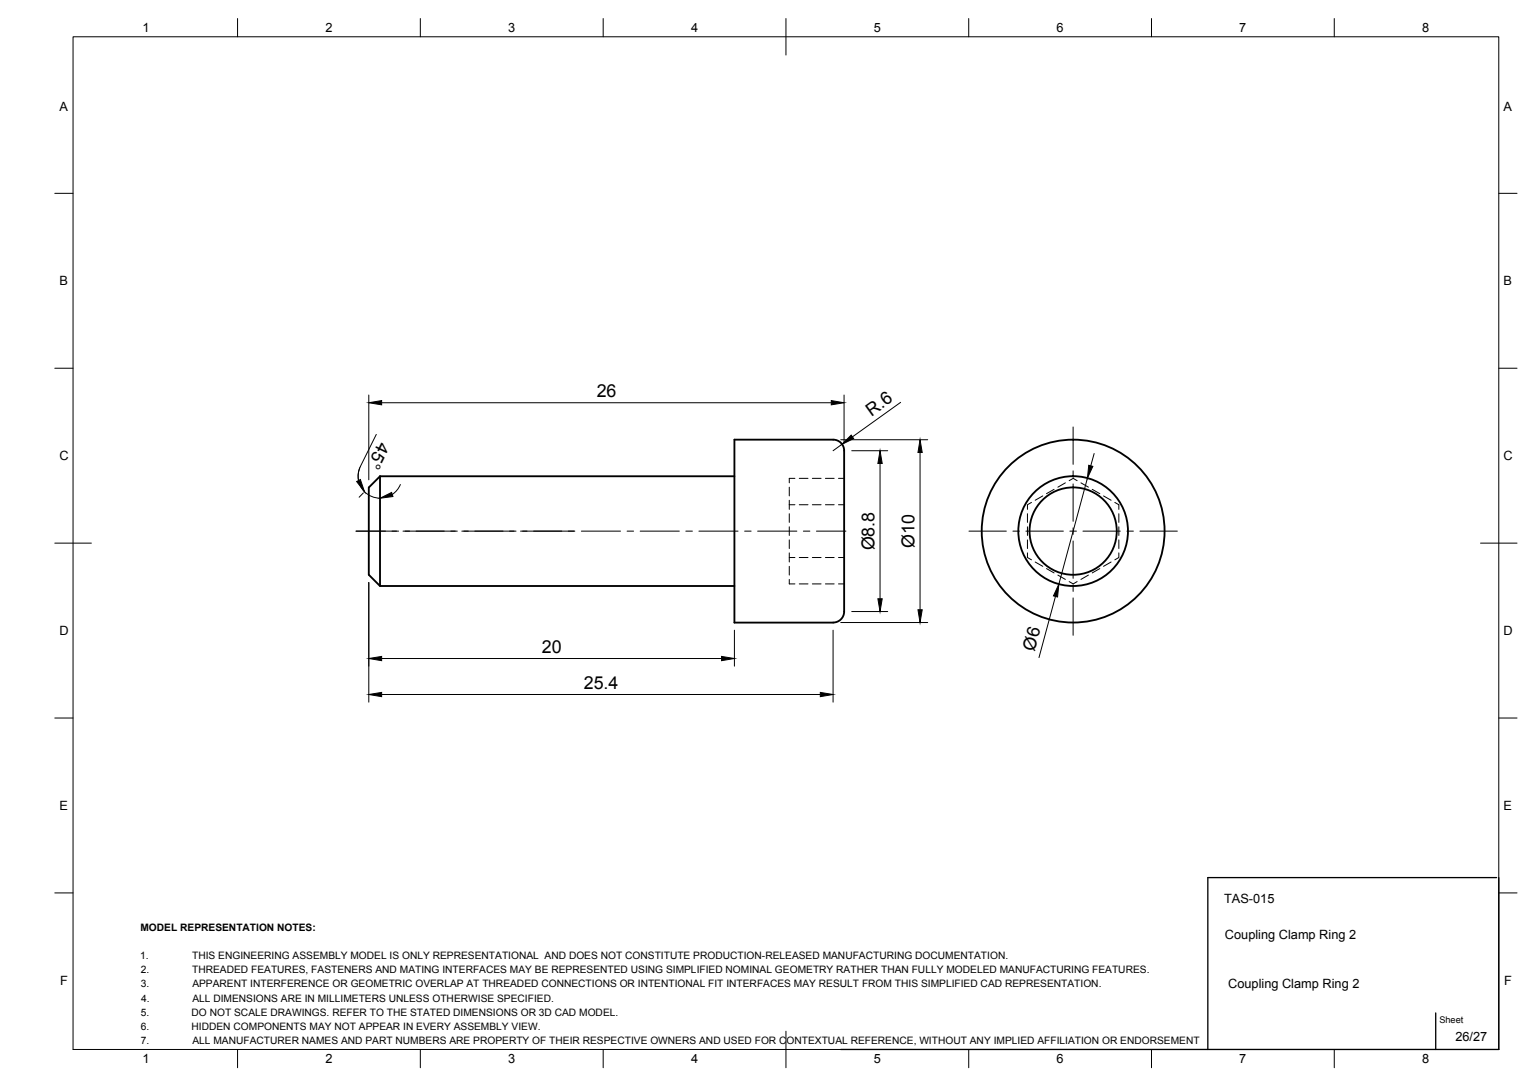
ISO-10303-21;
HEADER;
/* Generated by software containing ST-Developer
 * from STEP Tools, Inc. (www.steptools.com) 
 */

FILE_DESCRIPTION(
/* description */ ('STEP AP214'),
/* implementation_level */ '2;1');

FILE_NAME(
/* name */ 'Coupling Clamp Ring 2.step',
/* time_stamp */ '2026-11-15T14:49:54-08:00',
/* author */ (''),
/* organization */ (''),
/* preprocessor_version */ 'ST-DEVELOPER v20.2',
/* originating_system */ 'Autodesk Translation Framework v15.17.0.0',
/* authorisation */ '');

FILE_SCHEMA (('AUTOMOTIVE_DESIGN { 1 0 10303 214 3 1 1 }'));
ENDSEC;

DATA;
#10=MECHANICAL_DESIGN_GEOMETRIC_PRESENTATION_REPRESENTATION('',(#1123),#66721);
#81=TOROIDAL_SURFACE('',#28250,4.3999999999,0.6);
#556=CONICAL_SURFACE('',#28263,2.693275,0.785398163397448);
#1060=SHAPE_REPRESENTATION_RELATIONSHIP('SRR','None',#66923,#1091);
#1091=ADVANCED_BREP_SHAPE_REPRESENTATION('',(#1158),#66714);
#1123=STYLED_ITEM('',(#67095),#1158);
#1158=MANIFOLD_SOLID_BREP('Body1',#25689);
#1430=FACE_BOUND('',#5182,.T.);
#1431=FACE_BOUND('',#5186,.T.);
#2138=PLANE('',#28245);
#2139=PLANE('',#28253);
#2140=PLANE('',#28254);
#2141=PLANE('',#28255);
#2142=PLANE('',#28256);
#2143=PLANE('',#28257);
#2144=PLANE('',#28258);
#2145=PLANE('',#28259);
#2146=PLANE('',#28260);
#2147=PLANE('',#28261);
#3477=FACE_OUTER_BOUND('',#5181,.T.);
#3478=FACE_OUTER_BOUND('',#5183,.T.);
#3479=FACE_OUTER_BOUND('',#5184,.T.);
#3480=FACE_OUTER_BOUND('',#5185,.T.);
#3481=FACE_OUTER_BOUND('',#5187,.T.);
#3482=FACE_OUTER_BOUND('',#5188,.T.);
#3483=FACE_OUTER_BOUND('',#5189,.T.);
#3484=FACE_OUTER_BOUND('',#5190,.T.);
#3485=FACE_OUTER_BOUND('',#5191,.T.);
#3486=FACE_OUTER_BOUND('',#5192,.T.);
#3487=FACE_OUTER_BOUND('',#5193,.T.);
#3488=FACE_OUTER_BOUND('',#5194,.T.);
#3489=FACE_OUTER_BOUND('',#5195,.T.);
#3490=FACE_OUTER_BOUND('',#5196,.T.);
#5181=EDGE_LOOP('',(#22708));
#5182=EDGE_LOOP('',(#22709));
#5183=EDGE_LOOP('',(#22710,#22711,#22712,#22713));
#5184=EDGE_LOOP('',(#22714,#22715,#22716,#22717));
#5185=EDGE_LOOP('',(#22718));
#5186=EDGE_LOOP('',(#22719,#22720,#22721,#22722,#22723,#22724));
#5187=EDGE_LOOP('',(#22725,#22726,#22727,#22728,#22729,#22730));
#5188=EDGE_LOOP('',(#22731,#22732,#22733,#22734));
#5189=EDGE_LOOP('',(#22735,#22736,#22737,#22738));
#5190=EDGE_LOOP('',(#22739,#22740,#22741,#22742));
#5191=EDGE_LOOP('',(#22743,#22744,#22745,#22746));
#5192=EDGE_LOOP('',(#22747,#22748,#22749,#22750));
#5193=EDGE_LOOP('',(#22751,#22752,#22753,#22754));
#5194=EDGE_LOOP('',(#22755));
#5195=EDGE_LOOP('',(#22756,#22757,#22758,#22759));
#5196=EDGE_LOOP('',(#22760,#22761,#22762,#22763));
#7145=LINE('',#65140,#9134);
#7146=LINE('',#65149,#9135);
#7147=LINE('',#65151,#9136);
#7148=LINE('',#65153,#9137);
#7149=LINE('',#65155,#9138);
#7150=LINE('',#65157,#9139);
#7151=LINE('',#65158,#9140);
#7152=LINE('',#65162,#9141);
#7153=LINE('',#65164,#9142);
#7154=LINE('',#65166,#9143);
#7155=LINE('',#65168,#9144);
#7156=LINE('',#65170,#9145);
#7157=LINE('',#65171,#9146);
#7158=LINE('',#65173,#9147);
#7159=LINE('',#65174,#9148);
#7160=LINE('',#65176,#9149);
#7161=LINE('',#65178,#9150);
#7162=LINE('',#65180,#9151);
#7163=LINE('',#65182,#9152);
#7164=LINE('',#65190,#9153);
#7165=LINE('',#65192,#9154);
#9134=VECTOR('',#34834,5.);
#9135=VECTOR('',#34845,1000.);
#9136=VECTOR('',#34846,1000.);
#9137=VECTOR('',#34847,1000.);
#9138=VECTOR('',#34848,1000.);
#9139=VECTOR('',#34849,1000.);
#9140=VECTOR('',#34850,1000.);
#9141=VECTOR('',#34853,1000.);
#9142=VECTOR('',#34854,1000.);
#9143=VECTOR('',#34855,1000.);
#9144=VECTOR('',#34856,1000.);
#9145=VECTOR('',#34857,1000.);
#9146=VECTOR('',#34858,1000.);
#9147=VECTOR('',#34861,1000.);
#9148=VECTOR('',#34862,1000.);
#9149=VECTOR('',#34865,1000.);
#9150=VECTOR('',#34868,1000.);
#9151=VECTOR('',#34871,1000.);
#9152=VECTOR('',#34874,1000.);
#9153=VECTOR('',#34885,2.693275);
#9154=VECTOR('',#34888,3.);
#10452=CIRCLE('',#28246,5.);
#10453=CIRCLE('',#28247,3.);
#10454=CIRCLE('',#28249,5.);
#10455=CIRCLE('',#28251,0.6);
#10456=CIRCLE('',#28252,4.4);
#10457=CIRCLE('',#28262,2.38655);
#10458=CIRCLE('',#28264,3.);
#12621=VERTEX_POINT('',#65134);
#12622=VERTEX_POINT('',#65136);
#12623=VERTEX_POINT('',#65139);
#12624=VERTEX_POINT('',#65143);
#12625=VERTEX_POINT('',#65147);
#12626=VERTEX_POINT('',#65148);
#12627=VERTEX_POINT('',#65150);
#12628=VERTEX_POINT('',#65152);
#12629=VERTEX_POINT('',#65154);
#12630=VERTEX_POINT('',#65156);
#12631=VERTEX_POINT('',#65160);
#12632=VERTEX_POINT('',#65161);
#12633=VERTEX_POINT('',#65163);
#12634=VERTEX_POINT('',#65165);
#12635=VERTEX_POINT('',#65167);
#12636=VERTEX_POINT('',#65169);
#12637=VERTEX_POINT('',#65185);
#12638=VERTEX_POINT('',#65188);
#16047=EDGE_CURVE('',#12621,#12621,#10452,.T.);
#16048=EDGE_CURVE('',#12622,#12622,#10453,.T.);
#16049=EDGE_CURVE('',#12621,#12623,#7145,.T.);
#16050=EDGE_CURVE('',#12623,#12623,#10454,.T.);
#16051=EDGE_CURVE('',#12623,#12624,#10455,.T.);
#16052=EDGE_CURVE('',#12624,#12624,#10456,.T.);
#16053=EDGE_CURVE('',#12625,#12626,#7146,.T.);
#16054=EDGE_CURVE('',#12626,#12627,#7147,.T.);
#16055=EDGE_CURVE('',#12627,#12628,#7148,.T.);
#16056=EDGE_CURVE('',#12628,#12629,#7149,.T.);
#16057=EDGE_CURVE('',#12629,#12630,#7150,.T.);
#16058=EDGE_CURVE('',#12630,#12625,#7151,.T.);
#16059=EDGE_CURVE('',#12631,#12632,#7152,.T.);
#16060=EDGE_CURVE('',#12632,#12633,#7153,.T.);
#16061=EDGE_CURVE('',#12633,#12634,#7154,.T.);
#16062=EDGE_CURVE('',#12634,#12635,#7155,.T.);
#16063=EDGE_CURVE('',#12635,#12636,#7156,.T.);
#16064=EDGE_CURVE('',#12636,#12631,#7157,.T.);
#16065=EDGE_CURVE('',#12627,#12636,#7158,.T.);
#16066=EDGE_CURVE('',#12626,#12631,#7159,.T.);
#16067=EDGE_CURVE('',#12628,#12635,#7160,.T.);
#16068=EDGE_CURVE('',#12629,#12634,#7161,.T.);
#16069=EDGE_CURVE('',#12630,#12633,#7162,.T.);
#16070=EDGE_CURVE('',#12625,#12632,#7163,.T.);
#16071=EDGE_CURVE('',#12637,#12637,#10457,.T.);
#16072=EDGE_CURVE('',#12638,#12638,#10458,.T.);
#16073=EDGE_CURVE('',#12638,#12637,#7164,.T.);
#16074=EDGE_CURVE('',#12638,#12622,#7165,.T.);
#22708=ORIENTED_EDGE('',*,*,#16047,.T.);
#22709=ORIENTED_EDGE('',*,*,#16048,.T.);
#22710=ORIENTED_EDGE('',*,*,#16047,.F.);
#22711=ORIENTED_EDGE('',*,*,#16049,.T.);
#22712=ORIENTED_EDGE('',*,*,#16050,.T.);
#22713=ORIENTED_EDGE('',*,*,#16049,.F.);
#22714=ORIENTED_EDGE('',*,*,#16050,.F.);
#22715=ORIENTED_EDGE('',*,*,#16051,.T.);
#22716=ORIENTED_EDGE('',*,*,#16052,.T.);
#22717=ORIENTED_EDGE('',*,*,#16051,.F.);
#22718=ORIENTED_EDGE('',*,*,#16052,.F.);
#22719=ORIENTED_EDGE('',*,*,#16053,.T.);
#22720=ORIENTED_EDGE('',*,*,#16054,.T.);
#22721=ORIENTED_EDGE('',*,*,#16055,.T.);
#22722=ORIENTED_EDGE('',*,*,#16056,.T.);
#22723=ORIENTED_EDGE('',*,*,#16057,.T.);
#22724=ORIENTED_EDGE('',*,*,#16058,.T.);
#22725=ORIENTED_EDGE('',*,*,#16059,.T.);
#22726=ORIENTED_EDGE('',*,*,#16060,.T.);
#22727=ORIENTED_EDGE('',*,*,#16061,.T.);
#22728=ORIENTED_EDGE('',*,*,#16062,.T.);
#22729=ORIENTED_EDGE('',*,*,#16063,.T.);
#22730=ORIENTED_EDGE('',*,*,#16064,.T.);
#22731=ORIENTED_EDGE('',*,*,#16064,.F.);
#22732=ORIENTED_EDGE('',*,*,#16065,.F.);
#22733=ORIENTED_EDGE('',*,*,#16054,.F.);
#22734=ORIENTED_EDGE('',*,*,#16066,.T.);
#22735=ORIENTED_EDGE('',*,*,#16063,.F.);
#22736=ORIENTED_EDGE('',*,*,#16067,.F.);
#22737=ORIENTED_EDGE('',*,*,#16055,.F.);
#22738=ORIENTED_EDGE('',*,*,#16065,.T.);
#22739=ORIENTED_EDGE('',*,*,#16062,.F.);
#22740=ORIENTED_EDGE('',*,*,#16068,.F.);
#22741=ORIENTED_EDGE('',*,*,#16056,.F.);
#22742=ORIENTED_EDGE('',*,*,#16067,.T.);
#22743=ORIENTED_EDGE('',*,*,#16061,.F.);
#22744=ORIENTED_EDGE('',*,*,#16069,.F.);
#22745=ORIENTED_EDGE('',*,*,#16057,.F.);
#22746=ORIENTED_EDGE('',*,*,#16068,.T.);
#22747=ORIENTED_EDGE('',*,*,#16060,.F.);
#22748=ORIENTED_EDGE('',*,*,#16070,.F.);
#22749=ORIENTED_EDGE('',*,*,#16058,.F.);
#22750=ORIENTED_EDGE('',*,*,#16069,.T.);
#22751=ORIENTED_EDGE('',*,*,#16059,.F.);
#22752=ORIENTED_EDGE('',*,*,#16066,.F.);
#22753=ORIENTED_EDGE('',*,*,#16053,.F.);
#22754=ORIENTED_EDGE('',*,*,#16070,.T.);
#22755=ORIENTED_EDGE('',*,*,#16071,.T.);
#22756=ORIENTED_EDGE('',*,*,#16072,.T.);
#22757=ORIENTED_EDGE('',*,*,#16073,.T.);
#22758=ORIENTED_EDGE('',*,*,#16071,.F.);
#22759=ORIENTED_EDGE('',*,*,#16073,.F.);
#22760=ORIENTED_EDGE('',*,*,#16072,.F.);
#22761=ORIENTED_EDGE('',*,*,#16074,.T.);
#22762=ORIENTED_EDGE('',*,*,#16048,.F.);
#22763=ORIENTED_EDGE('',*,*,#16074,.F.);
#24146=CYLINDRICAL_SURFACE('',#28248,5.);
#24147=CYLINDRICAL_SURFACE('',#28265,3.);
#25430=ADVANCED_FACE('',(#3477,#1430),#2138,.T.);
#25431=ADVANCED_FACE('',(#3478),#24146,.T.);
#25432=ADVANCED_FACE('',(#3479),#81,.T.);
#25433=ADVANCED_FACE('',(#3480,#1431),#2139,.T.);
#25434=ADVANCED_FACE('',(#3481),#2140,.F.);
#25435=ADVANCED_FACE('',(#3482),#2141,.F.);
#25436=ADVANCED_FACE('',(#3483),#2142,.F.);
#25437=ADVANCED_FACE('',(#3484),#2143,.F.);
#25438=ADVANCED_FACE('',(#3485),#2144,.F.);
#25439=ADVANCED_FACE('',(#3486),#2145,.F.);
#25440=ADVANCED_FACE('',(#3487),#2146,.F.);
#25441=ADVANCED_FACE('',(#3488),#2147,.T.);
#25442=ADVANCED_FACE('',(#3489),#556,.T.);
#25443=ADVANCED_FACE('',(#3490),#24147,.T.);
#25689=CLOSED_SHELL('',(#25430,#25431,#25432,#25433,#25434,#25435,#25436,
#25437,#25438,#25439,#25440,#25441,#25442,#25443));
#28244=AXIS2_PLACEMENT_3D('',#65132,#34824,#34825);
#28245=AXIS2_PLACEMENT_3D('',#65133,#34826,#34827);
#28246=AXIS2_PLACEMENT_3D('',#65135,#34828,#34829);
#28247=AXIS2_PLACEMENT_3D('',#65137,#34830,#34831);
#28248=AXIS2_PLACEMENT_3D('',#65138,#34832,#34833);
#28249=AXIS2_PLACEMENT_3D('',#65141,#34835,#34836);
#28250=AXIS2_PLACEMENT_3D('',#65142,#34837,#34838);
#28251=AXIS2_PLACEMENT_3D('',#65144,#34839,#34840);
#28252=AXIS2_PLACEMENT_3D('',#65145,#34841,#34842);
#28253=AXIS2_PLACEMENT_3D('',#65146,#34843,#34844);
#28254=AXIS2_PLACEMENT_3D('',#65159,#34851,#34852);
#28255=AXIS2_PLACEMENT_3D('',#65172,#34859,#34860);
#28256=AXIS2_PLACEMENT_3D('',#65175,#34863,#34864);
#28257=AXIS2_PLACEMENT_3D('',#65177,#34866,#34867);
#28258=AXIS2_PLACEMENT_3D('',#65179,#34869,#34870);
#28259=AXIS2_PLACEMENT_3D('',#65181,#34872,#34873);
#28260=AXIS2_PLACEMENT_3D('',#65183,#34875,#34876);
#28261=AXIS2_PLACEMENT_3D('',#65184,#34877,#34878);
#28262=AXIS2_PLACEMENT_3D('',#65186,#34879,#34880);
#28263=AXIS2_PLACEMENT_3D('',#65187,#34881,#34882);
#28264=AXIS2_PLACEMENT_3D('',#65189,#34883,#34884);
#28265=AXIS2_PLACEMENT_3D('',#65191,#34886,#34887);
#34824=DIRECTION('axis',(0.,0.,1.));
#34825=DIRECTION('refdir',(1.,0.,0.));
#34826=DIRECTION('center_axis',(0.,-0.707106781186548,-0.707106781186548));
#34827=DIRECTION('ref_axis',(0.,-0.707106781186548,0.707106781186548));
#34828=DIRECTION('center_axis',(0.,-0.707106781186548,-0.707106781186548));
#34829=DIRECTION('ref_axis',(-1.,0.,0.));
#34830=DIRECTION('center_axis',(0.,0.707106781186548,0.707106781186548));
#34831=DIRECTION('ref_axis',(-1.,0.,0.));
#34832=DIRECTION('center_axis',(0.,-0.707106781186548,-0.707106781186548));
#34833=DIRECTION('ref_axis',(-1.,0.,0.));
#34834=DIRECTION('',(0.,0.707106781186547,0.707106781186547));
#34835=DIRECTION('center_axis',(0.,-0.707106781186548,-0.707106781186548));
#34836=DIRECTION('ref_axis',(-1.,0.,0.));
#34837=DIRECTION('center_axis',(0.,-0.707106781186548,-0.707106781186548));
#34838=DIRECTION('ref_axis',(-1.,0.,0.));
#34839=DIRECTION('center_axis',(-7.85046229357589E-17,-0.707106781186548,
0.707106781186548));
#34840=DIRECTION('ref_axis',(1.,0.,1.11022302464736E-16));
#34841=DIRECTION('center_axis',(0.,-0.707106781186548,-0.707106781186548));
#34842=DIRECTION('ref_axis',(-1.,0.,0.));
#34843=DIRECTION('center_axis',(-2.27272746077357E-11,0.707106781186548,
0.707106781186548));
#34844=DIRECTION('ref_axis',(1.,-1.16819139994433E-27,3.21412199860375E-11));
#34845=DIRECTION('',(0.,-0.707106781186547,0.707106781186547));
#34846=DIRECTION('',(-0.866025403795548,-0.353553390593585,0.35355339056575));
#34847=DIRECTION('',(-0.866025403795548,0.35355339056575,-0.353553390593585));
#34848=DIRECTION('',(0.,0.707106781186547,-0.707106781186547));
#34849=DIRECTION('',(0.866025403795548,0.353553390593585,-0.35355339056575));
#34850=DIRECTION('',(0.866025403795548,-0.35355339056575,0.353553390593585));
#34851=DIRECTION('center_axis',(0.,-0.707106781186547,-0.707106781186548));
#34852=DIRECTION('ref_axis',(0.,-0.707106781186548,0.707106781186547));
#34853=DIRECTION('',(0.,0.707106781186548,-0.707106781186547));
#34854=DIRECTION('',(-0.866025403795548,0.353553390579667,-0.353553390579667));
#34855=DIRECTION('',(-0.866025403795548,-0.353553390579667,0.353553390579667));
#34856=DIRECTION('',(0.,-0.707106781186548,0.707106781186547));
#34857=DIRECTION('',(0.866025403795548,-0.353553390579667,0.353553390579667));
#34858=DIRECTION('',(0.866025403795548,0.353553390579667,-0.353553390579667));
#34859=DIRECTION('center_axis',(0.499999999980758,-0.61237243570365,0.61237243570365));
#34860=DIRECTION('ref_axis',(-0.774596669257382,-0.632455532014204,1.19590756914335E-17));
#34861=DIRECTION('',(0.,-0.707106781186547,-0.707106781186548));
#34862=DIRECTION('',(0.,-0.707106781186547,-0.707106781186548));
#34863=DIRECTION('center_axis',(-0.499999999980758,-0.61237243570365,0.61237243570365));
#34864=DIRECTION('ref_axis',(-0.774596669257382,0.632455532014204,-1.19590756914335E-17));
#34865=DIRECTION('',(0.,-0.707106781186547,-0.707106781186548));
#34866=DIRECTION('center_axis',(-1.,0.,0.));
#34867=DIRECTION('ref_axis',(0.,0.,1.));
#34868=DIRECTION('',(0.,-0.707106781186547,-0.707106781186548));
#34869=DIRECTION('center_axis',(-0.499999999980758,0.61237243570365,-0.61237243570365));
#34870=DIRECTION('ref_axis',(-0.774596669257382,-1.17004406563443E-17,0.632455532014204));
#34871=DIRECTION('',(0.,-0.707106781186547,-0.707106781186548));
#34872=DIRECTION('center_axis',(0.499999999980758,0.61237243570365,-0.61237243570365));
#34873=DIRECTION('ref_axis',(-0.774596669257382,1.17004406563443E-17,-0.632455532014204));
#34874=DIRECTION('',(0.,-0.707106781186547,-0.707106781186548));
#34875=DIRECTION('center_axis',(1.,0.,0.));
#34876=DIRECTION('ref_axis',(0.,1.,0.));
#34877=DIRECTION('center_axis',(0.,-0.707106781186548,-0.707106781186548));
#34878=DIRECTION('ref_axis',(0.,-0.707106781186548,0.707106781186548));
#34879=DIRECTION('center_axis',(0.,-0.707106781186548,-0.707106781186548));
#34880=DIRECTION('ref_axis',(-1.,0.,0.));
#34881=DIRECTION('center_axis',(0.,0.707106781186548,0.707106781186548));
#34882=DIRECTION('ref_axis',(-1.,0.,0.));
#34883=DIRECTION('center_axis',(0.,-0.707106781186548,-0.707106781186548));
#34884=DIRECTION('ref_axis',(-1.,0.,0.));
#34885=DIRECTION('',(-0.707106781186547,-0.5,-0.5));
#34886=DIRECTION('center_axis',(0.,-0.707106781186548,-0.707106781186548));
#34887=DIRECTION('ref_axis',(-1.,0.,0.));
#34888=DIRECTION('',(0.,0.707106781186548,0.707106781186548));
#65132=CARTESIAN_POINT('',(0.,0.,0.));
#65133=CARTESIAN_POINT('Origin',(-26.5,22.6274169980807,-5.65685424941929));
#65134=CARTESIAN_POINT('',(-19.,22.6274169980807,-5.65685424941929));
#65135=CARTESIAN_POINT('Origin',(-24.,22.6274169980807,-5.65685424941929));
#65136=CARTESIAN_POINT('',(-21.,22.6274169980807,-5.65685424941928));
#65137=CARTESIAN_POINT('Origin',(-24.,22.6274169980807,-5.65685424941928));
#65138=CARTESIAN_POINT('Origin',(-24.,24.5366053072844,-3.74766594021561));
#65139=CARTESIAN_POINT('',(-19.,26.4457936164881,-1.83847763101193));
#65140=CARTESIAN_POINT('',(-19.,24.5366053072844,-3.74766594021561));
#65141=CARTESIAN_POINT('Origin',(-24.,26.4457936164881,-1.83847763101193));
#65142=CARTESIAN_POINT('Origin',(-24.,26.4457936164174,-1.83847763108264));
#65143=CARTESIAN_POINT('',(-19.6,26.8700576851293,-1.41421356237071));
#65144=CARTESIAN_POINT('Origin',(-19.6000000001,26.4457936164174,-1.83847763108264));
#65145=CARTESIAN_POINT('Origin',(-24.,26.8700576851293,-1.41421356237071));
#65146=CARTESIAN_POINT('Origin',(-26.2,26.8700576851646,-1.41421356233536));
#65147=CARTESIAN_POINT('',(-21.5,27.890678411278,-2.434834288578));
#65148=CARTESIAN_POINT('',(-21.5,25.849436958922,-0.393592836222004));
#65149=CARTESIAN_POINT('',(-21.5,26.8700576852402,-1.41421356225982));
#65150=CARTESIAN_POINT('',(-24.,24.8288162328147,0.627027889885282));
#65151=CARTESIAN_POINT('',(-23.5750000000476,25.0023217562335,0.453522366466486));
#65152=CARTESIAN_POINT('',(-26.5,25.849436958922,-0.393592836222004));
#65153=CARTESIAN_POINT('',(-26.0749999999947,25.6759314354816,-0.220087312781607));
#65154=CARTESIAN_POINT('',(-26.5,27.890678411278,-2.434834288578));
#65155=CARTESIAN_POINT('',(-26.5,26.6149025036153,-1.15905838079568));
#65156=CARTESIAN_POINT('',(-24.,28.9112991373853,-3.45545501468528));
#65157=CARTESIAN_POINT('',(-26.0749999999947,28.0641839347184,-2.60833981201839));
#65158=CARTESIAN_POINT('',(-23.5750000000476,28.7377936139665,-3.28194949126649));
#65159=CARTESIAN_POINT('Origin',(-24.,24.7487373415404,-3.53553390595964));
#65160=CARTESIAN_POINT('',(-21.5,23.7281166153624,-2.51491317978165));
#65161=CARTESIAN_POINT('',(-21.5,25.7693580677184,-4.55615463213764));
#65162=CARTESIAN_POINT('',(-21.5,25.7693580677184,-4.55615463213764));
#65163=CARTESIAN_POINT('',(-24.,26.7899787938256,-5.57677535824492));
#65164=CARTESIAN_POINT('',(-24.,26.7899787938256,-5.57677535824492));
#65165=CARTESIAN_POINT('',(-26.5,25.7693580677184,-4.55615463213764));
#65166=CARTESIAN_POINT('',(-26.5,25.7693580677184,-4.55615463213764));
#65167=CARTESIAN_POINT('',(-26.5,23.7281166153624,-2.51491317978165));
#65168=CARTESIAN_POINT('',(-26.5,24.7487373415404,-3.53553390595964));
#65169=CARTESIAN_POINT('',(-24.,22.7074958892551,-1.49429245367436));
#65170=CARTESIAN_POINT('',(-24.,22.7074958892551,-1.49429245367436));
#65171=CARTESIAN_POINT('',(-21.5,23.7281166153624,-2.51491317978165));
#65172=CARTESIAN_POINT('Origin',(-22.75,25.3391265958684,0.116717526831639));
#65173=CARTESIAN_POINT('',(-24.,24.8288162328147,0.627027889885282));
#65174=CARTESIAN_POINT('',(-21.5,25.849436958922,-0.393592836222004));
#65175=CARTESIAN_POINT('Origin',(-25.25,25.3391265958684,0.116717526831639));
#65176=CARTESIAN_POINT('',(-26.5,25.849436958922,-0.393592836222004));
#65177=CARTESIAN_POINT('Origin',(-26.5,26.359747322011,-0.903903199311002));
#65178=CARTESIAN_POINT('',(-26.5,27.890678411278,-2.434834288578));
#65179=CARTESIAN_POINT('Origin',(-25.25,28.4009887743316,-2.94514465163164));
#65180=CARTESIAN_POINT('',(-24.,28.9112991373853,-3.45545501468528));
#65181=CARTESIAN_POINT('Origin',(-22.75,28.4009887743316,-2.94514465163164));
#65182=CARTESIAN_POINT('',(-21.5,27.890678411278,-2.434834288578));
#65183=CARTESIAN_POINT('Origin',(-21.5,26.8700576851,-1.4142135624));
#65184=CARTESIAN_POINT('Origin',(-25.193275,8.48528137426905,-19.798989873231));
#65185=CARTESIAN_POINT('',(-21.61345,8.48528137426905,-19.7989898732309));
#65186=CARTESIAN_POINT('Origin',(-24.,8.48528137426905,-19.798989873231));
#65187=CARTESIAN_POINT('Origin',(-24.,8.70216870172849,-19.5821025457715));
#65188=CARTESIAN_POINT('',(-21.,8.91905602918794,-19.3652152183121));
#65189=CARTESIAN_POINT('Origin',(-24.,8.91905602918794,-19.3652152183121));
#65190=CARTESIAN_POINT('',(-21.306725,8.70216870172849,-19.5821025457715));
#65191=CARTESIAN_POINT('Origin',(-24.,15.773236513594,-12.511034733906));
#65192=CARTESIAN_POINT('',(-21.,15.773236513594,-12.511034733906));
#66673=UNCERTAINTY_MEASURE_WITH_UNIT(LENGTH_MEASURE(0.01),#66722,
'DISTANCE_ACCURACY_VALUE',
'Maximum model space distance between geometric entities at asserted c
onnectivities');
#66680=UNCERTAINTY_MEASURE_WITH_UNIT(LENGTH_MEASURE(0.01),#66722,
'DISTANCE_ACCURACY_VALUE',
'Maximum model space distance between geometric entities at asserted c
onnectivities');
#66714=(
GEOMETRIC_REPRESENTATION_CONTEXT(3)
GLOBAL_UNCERTAINTY_ASSIGNED_CONTEXT((#66673))
GLOBAL_UNIT_ASSIGNED_CONTEXT((#66722,#66724,#66725))
REPRESENTATION_CONTEXT('','3D')
);
#66721=(
GEOMETRIC_REPRESENTATION_CONTEXT(3)
GLOBAL_UNCERTAINTY_ASSIGNED_CONTEXT((#66680))
GLOBAL_UNIT_ASSIGNED_CONTEXT((#66722,#66724,#66725))
REPRESENTATION_CONTEXT('','3D')
);
#66722=(
LENGTH_UNIT()
NAMED_UNIT(*)
SI_UNIT(.MILLI.,.METRE.)
);
#66724=(
NAMED_UNIT(*)
PLANE_ANGLE_UNIT()
SI_UNIT($,.RADIAN.)
);
#66725=(
NAMED_UNIT(*)
SI_UNIT($,.STERADIAN.)
SOLID_ANGLE_UNIT()
);
#66759=SHAPE_DEFINITION_REPRESENTATION(#66819,#66923);
#66819=PRODUCT_DEFINITION_SHAPE('',$,#66964);
#66923=SHAPE_REPRESENTATION('',(#28244),#66714);
#66930=PRODUCT_DEFINITION_CONTEXT('part definition',#67052,'design');
#66964=PRODUCT_DEFINITION('Coupling Clamp Ring 2',
'Coupling Clamp Ring 2',#67004,#66930);
#67004=PRODUCT_DEFINITION_FORMATION('',$,#67087);
#67052=APPLICATION_CONTEXT(
'Core Data for Automotive Mechanical Design Process');
#67053=PRODUCT_CONTEXT('part definition',#67052,'mechanical');
#67087=PRODUCT('Coupling Clamp Ring 2','Coupling Clamp Ring 2',$,(#67053));
#67095=PRESENTATION_STYLE_ASSIGNMENT((#67097));
#67097=SURFACE_STYLE_USAGE(.BOTH.,#67099);
#67099=SURFACE_SIDE_STYLE('',(#67101));
#67101=SURFACE_STYLE_FILL_AREA(#67103);
#67103=FILL_AREA_STYLE('Opaque(202,209,238)',(#67105));
#67105=FILL_AREA_STYLE_COLOUR('Opaque(202,209,238)',#67107);
#67107=COLOUR_RGB('Opaque(202,209,238)',0.792156862745098,0.819607843137255,
0.933333333333333);
ENDSEC;
END-ISO-10303-21;
